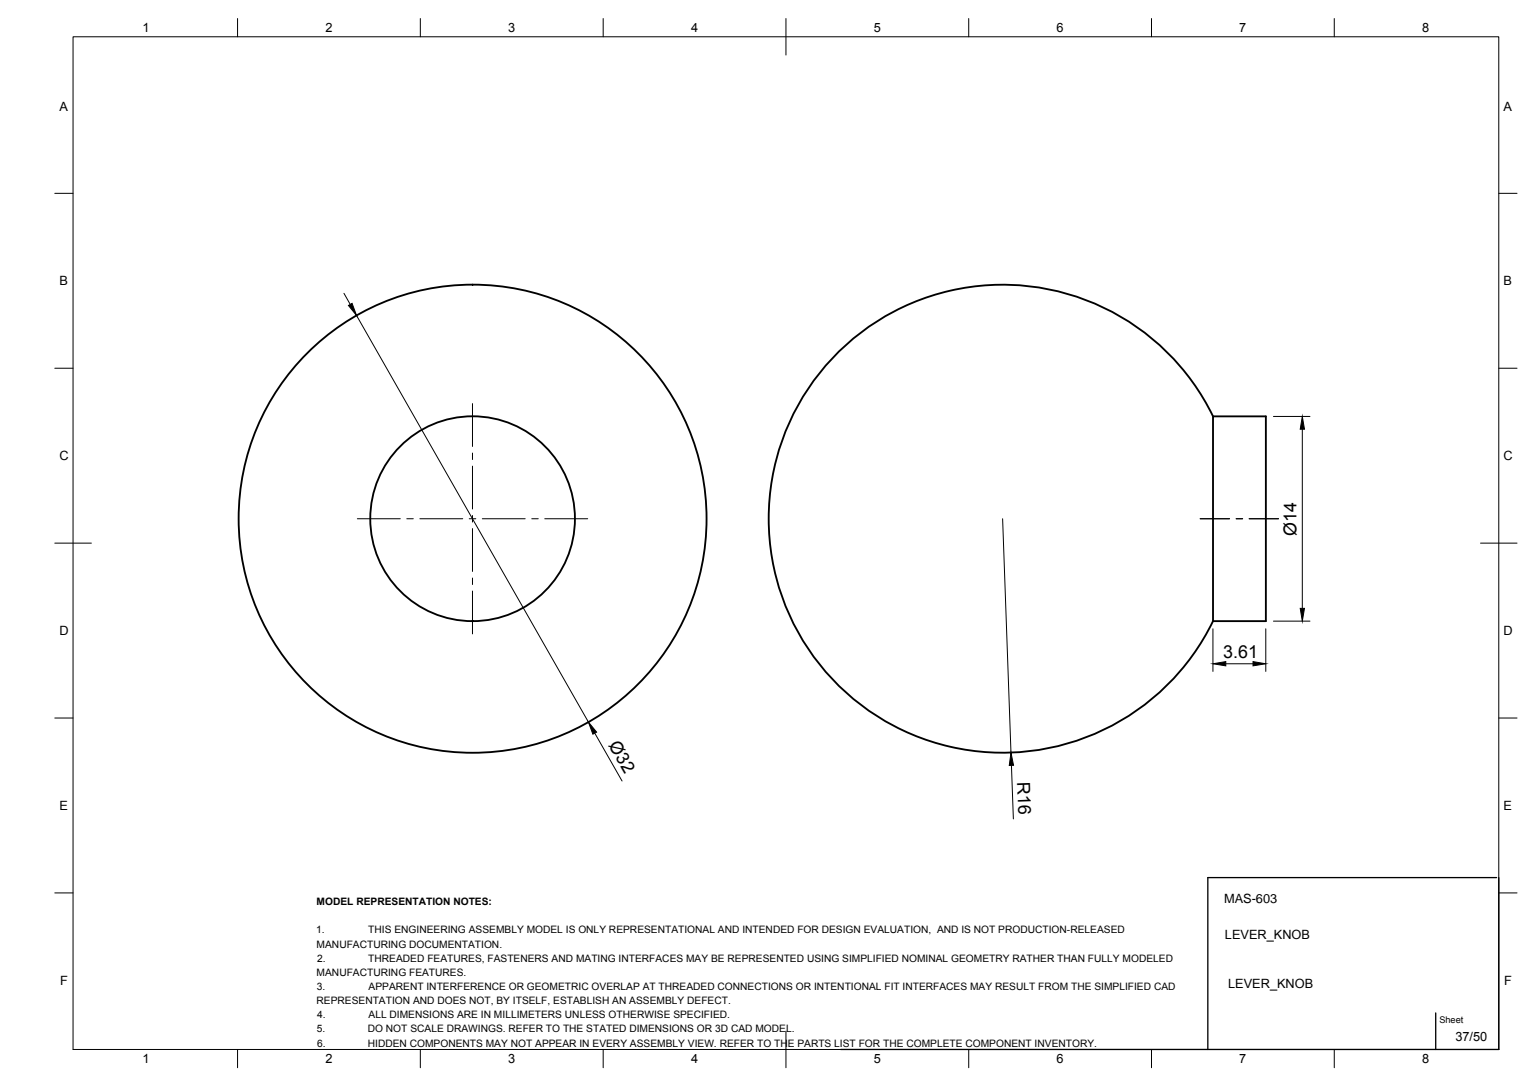
ISO-10303-21;
HEADER;
FILE_DESCRIPTION((''),'2;1');
FILE_NAME('LEVER_KNOB.step','2026-10-01T22:06:14-07:00',(''),(''),'','','');
FILE_SCHEMA (('AUTOMOTIVE_DESIGN { 1 0 10303 214 3 1 1 }'));
ENDSEC;
DATA;
#10=MECHANICAL_DESIGN_GEOMETRIC_PRESENTATION_REPRESENTATION('',(#1010),#50440);
#727=SPHERICAL_SURFACE('',#30930,1.6) ;
#917=SHAPE_REPRESENTATION_RELATIONSHIP('SRR','None',#50650,#962) ;
#962=ADVANCED_BREP_SHAPE_REPRESENTATION('',(#1065),#50419) ;
#1010=STYLED_ITEM('',(#50888),#1065) ;
#1065=MANIFOLD_SOLID_BREP('LEVER_KNOB',#28677) ;
#2228=PLANE('',#30929) ;
#3412=FACE_OUTER_BOUND('',#5230,.T.) ;
#3413=FACE_OUTER_BOUND('',#5231,.T.) ;
#3414=FACE_OUTER_BOUND('',#5232,.T.) ;
#5230=EDGE_LOOP('',(#24085,#24086,#24087,#24088)) ;
#5231=EDGE_LOOP('',(#24089)) ;
#5232=EDGE_LOOP('',(#24090,#24091,#24092)) ;
#7878=LINE('',#47179,#10350) ;
#10350=VECTOR('',#37959,0.7) ;
#11232=CIRCLE('',#30927,0.700000000000003) ;
#11233=CIRCLE('',#30928,0.7) ;
#11234=CIRCLE('',#30931,1.6) ;
#13676=VERTEX_POINT('',#47176) ;
#13677=VERTEX_POINT('',#47178) ;
#13678=VERTEX_POINT('',#47183) ;
#17308=EDGE_CURVE('',#13676,#13676,#11232,.T.) ;
#17309=EDGE_CURVE('',#13676,#13677,#7878,.T.) ;
#17310=EDGE_CURVE('',#13677,#13677,#11233,.T.) ;
#17311=EDGE_CURVE('',#13678,#13676,#11234,.T.) ;
#24085=ORIENTED_EDGE('',*,*,#17308,.F.) ;
#24086=ORIENTED_EDGE('',*,*,#17309,.T.) ;
#24087=ORIENTED_EDGE('',*,*,#17310,.F.) ;
#24088=ORIENTED_EDGE('',*,*,#17309,.F.) ;
#24089=ORIENTED_EDGE('',*,*,#17310,.T.) ;
#24090=ORIENTED_EDGE('',*,*,#17308,.T.) ;
#24091=ORIENTED_EDGE('',*,*,#17311,.F.) ;
#24092=ORIENTED_EDGE('',*,*,#17311,.T.) ;
#26869=CYLINDRICAL_SURFACE('',#30926,0.7) ;
#28147=ADVANCED_FACE('',(#3412),#26869,.T.) ;
#28148=ADVANCED_FACE('',(#3413),#2228,.T.) ;
#28149=ADVANCED_FACE('',(#3414),#727,.T.) ;
#28677=CLOSED_SHELL('',(#28147,#28148,#28149)) ;
#30925=AXIS2_PLACEMENT_3D('',#47174,#37953,#37954) ;
#30926=AXIS2_PLACEMENT_3D('',#47175,#37955,#37956) ;
#30927=AXIS2_PLACEMENT_3D('',#47177,#37957,#37958) ;
#30928=AXIS2_PLACEMENT_3D('',#47180,#37960,#37961) ;
#30929=AXIS2_PLACEMENT_3D('',#47181,#37962,#37963) ;
#30930=AXIS2_PLACEMENT_3D('',#47182,#37964,#37965) ;
#30931=AXIS2_PLACEMENT_3D('',#47184,#37966,#37967) ;
#37953=DIRECTION('axis',(0.,0.,1.)) ;
#37954=DIRECTION('refdir',(1.,0.,0.)) ;
#37955=DIRECTION('center_axis',(0.,0.,1.)) ;
#37956=DIRECTION('ref_axis',(1.,0.,0.)) ;
#37957=DIRECTION('center_axis',(0.,0.,1.)) ;
#37958=DIRECTION('ref_axis',(1.,0.,0.)) ;
#37959=DIRECTION('',(0.,0.,-1.)) ;
#37960=DIRECTION('center_axis',(0.,0.,-1.)) ;
#37961=DIRECTION('ref_axis',(1.,0.,0.)) ;
#37962=DIRECTION('center_axis',(0.,0.,-1.)) ;
#37963=DIRECTION('ref_axis',(-1.,0.,0.)) ;
#37964=DIRECTION('center_axis',(0.,0.,1.)) ;
#37965=DIRECTION('ref_axis',(1.,0.,0.)) ;
#37966=DIRECTION('center_axis',(0.,-1.,0.)) ;
#37967=DIRECTION('ref_axis',(-1.,0.,0.)) ;
#47174=CARTESIAN_POINT('',(0.,0.,0.)) ;
#47175=CARTESIAN_POINT('Origin',(-53.,19.,104.3)) ;
#47176=CARTESIAN_POINT('',(-53.7,19.,104.361250543006)) ;
#47177=CARTESIAN_POINT('Origin',(-53.,19.,104.361250543006)) ;
#47178=CARTESIAN_POINT('',(-53.7,19.,104.)) ;
#47179=CARTESIAN_POINT('',(-53.7,19.,104.3)) ;
#47180=CARTESIAN_POINT('Origin',(-53.,19.,104.)) ;
#47181=CARTESIAN_POINT('Origin',(-53.,19.,104.)) ;
#47182=CARTESIAN_POINT('Origin',(-53.,19.,105.8)) ;
#47183=CARTESIAN_POINT('',(-53.,19.,107.4)) ;
#47184=CARTESIAN_POINT('Origin',(-53.,19.,105.8)) ;
#50366=UNCERTAINTY_MEASURE_WITH_UNIT(LENGTH_MEASURE(0.001),#50441,
'DISTANCE_ACCURACY_VALUE',
'Maximum model space distance between geometric entities at asserted c
onnectivities') ;
#50387=UNCERTAINTY_MEASURE_WITH_UNIT(LENGTH_MEASURE(0.001),#50441,
'DISTANCE_ACCURACY_VALUE',
'Maximum model space distance between geometric entities at asserted c
onnectivities') ;
#50419=(
GEOMETRIC_REPRESENTATION_CONTEXT(3)
GLOBAL_UNCERTAINTY_ASSIGNED_CONTEXT((#50366))
GLOBAL_UNIT_ASSIGNED_CONTEXT((#50441,#50443,#50444))
REPRESENTATION_CONTEXT('','3D')
) ;
#50440=(
GEOMETRIC_REPRESENTATION_CONTEXT(3)
GLOBAL_UNCERTAINTY_ASSIGNED_CONTEXT((#50387))
GLOBAL_UNIT_ASSIGNED_CONTEXT((#50441,#50443,#50444))
REPRESENTATION_CONTEXT('','3D')
) ;
#50441=(
LENGTH_UNIT()
NAMED_UNIT(*)
SI_UNIT(.CENTI.,.METRE.)
) ;
#50443=(
NAMED_UNIT(*)
PLANE_ANGLE_UNIT()
SI_UNIT($,.RADIAN.)
) ;
#50444=(
NAMED_UNIT(*)
SI_UNIT($,.STERADIAN.)
SOLID_ANGLE_UNIT()
) ;
#50476=SHAPE_DEFINITION_REPRESENTATION(#50552,#50650) ;
#50552=PRODUCT_DEFINITION_SHAPE('',$,#50703) ;
#50650=SHAPE_REPRESENTATION('',(#30925),#50419) ;
#50671=PRODUCT_DEFINITION_CONTEXT('part definition',#50829,'design') ;
#50703=PRODUCT_DEFINITION('LEVER_KNOB','LEVER_KNOB',#50755,
#50671) ;
#50755=PRODUCT_DEFINITION_FORMATION('',$,#50862) ;
#50829=APPLICATION_CONTEXT(
'Core Data for Automotive Mechanical Design Process') ;
#50830=PRODUCT_CONTEXT('part definition',#50829,'mechanical') ;
#50862=PRODUCT('LEVER_KNOB','LEVER_KNOB',$,(#50830)) ;
#50888=PRESENTATION_STYLE_ASSIGNMENT((#50895)) ;
#50895=SURFACE_STYLE_USAGE(.BOTH.,#50902) ;
#50902=SURFACE_SIDE_STYLE('',(#50909)) ;
#50909=SURFACE_STYLE_FILL_AREA(#50916) ;
#50916=FILL_AREA_STYLE('Rubber - Soft',(#50923)) ;
#50923=FILL_AREA_STYLE_COLOUR('Rubber - Soft',#50930) ;
#50930=COLOUR_RGB('Rubber - Soft', 0.40784314, 0.44705882, 0.49803922) ;
ENDSEC;
END-ISO-10303-21;
